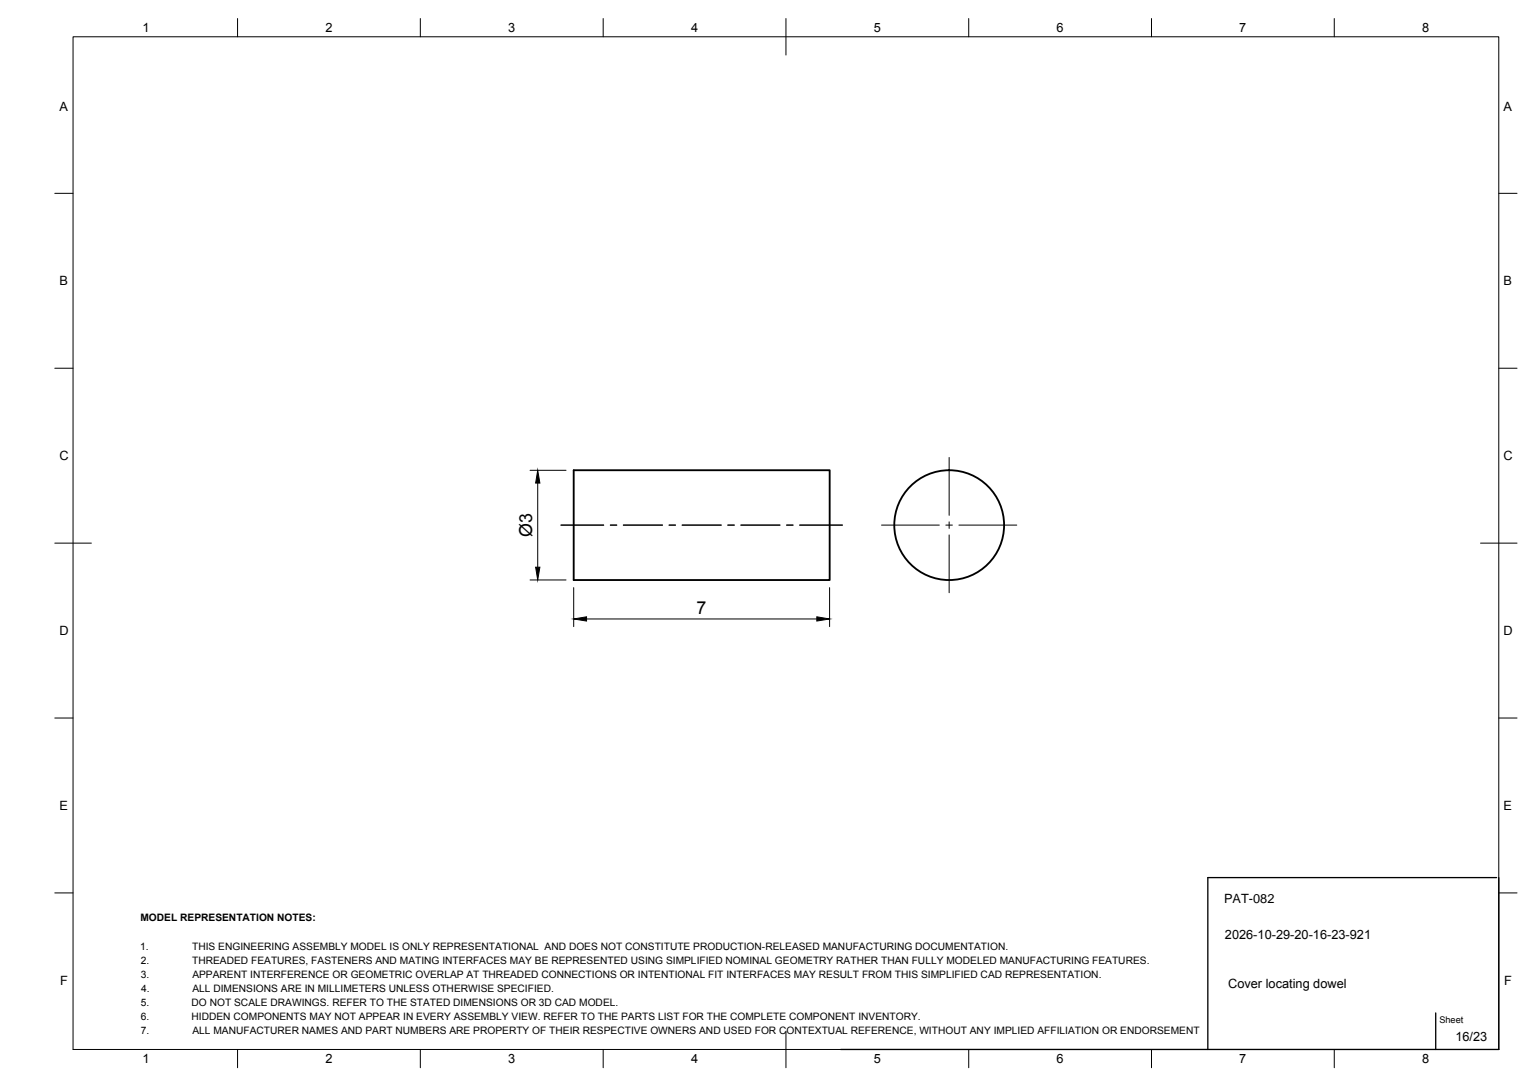
ISO-10303-21;
HEADER;
/* Generated by software containing ST-Developer
 * from STEP Tools, Inc. (www.steptools.com) 
 */

FILE_DESCRIPTION(
/* description */ ('PAT-082'),
/* implementation_level */ '2;1');

FILE_NAME(
/* name */ 'Cover locating dowel.step',
/* time_stamp */ '2026-10-29T20:16:13-07:00',
/* author */ (''),
/* organization */ (''),
/* preprocessor_version */ 'ST-DEVELOPER v20.2',
/* originating_system */ 'Autodesk Translation Framework v15.17.0.0',
/* authorisation */ '');

FILE_SCHEMA (('AUTOMOTIVE_DESIGN { 1 0 10303 214 3 1 1 }'));
ENDSEC;

DATA;
#10=MECHANICAL_DESIGN_GEOMETRIC_PRESENTATION_REPRESENTATION('',(#254),#8266);
#210=SHAPE_REPRESENTATION_RELATIONSHIP('SRR','None',#8372,#232);
#232=ADVANCED_BREP_SHAPE_REPRESENTATION('',(#276),#8256);
#254=STYLED_ITEM('',(#8530),#276);
#276=MANIFOLD_SOLID_BREP('Body1',#4594);
#504=PLANE('',#5182);
#505=PLANE('',#5183);
#741=FACE_OUTER_BOUND('',#1114,.T.);
#742=FACE_OUTER_BOUND('',#1115,.T.);
#743=FACE_OUTER_BOUND('',#1116,.T.);
#1114=EDGE_LOOP('',(#3842,#3843,#3844,#3845));
#1115=EDGE_LOOP('',(#3846));
#1116=EDGE_LOOP('',(#3847));
#1455=LINE('',#7761,#1810);
#1810=VECTOR('',#6266,0.15);
#2091=CIRCLE('',#5180,0.15);
#2092=CIRCLE('',#5181,0.15);
#2397=VERTEX_POINT('',#7758);
#2398=VERTEX_POINT('',#7760);
#2897=EDGE_CURVE('',#2397,#2397,#2091,.T.);
#2898=EDGE_CURVE('',#2397,#2398,#1455,.T.);
#2899=EDGE_CURVE('',#2398,#2398,#2092,.T.);
#3842=ORIENTED_EDGE('',*,*,#2897,.F.);
#3843=ORIENTED_EDGE('',*,*,#2898,.T.);
#3844=ORIENTED_EDGE('',*,*,#2899,.T.);
#3845=ORIENTED_EDGE('',*,*,#2898,.F.);
#3846=ORIENTED_EDGE('',*,*,#2897,.T.);
#3847=ORIENTED_EDGE('',*,*,#2899,.F.);
#4290=CYLINDRICAL_SURFACE('',#5179,0.15);
#4480=ADVANCED_FACE('',(#741),#4290,.T.);
#4481=ADVANCED_FACE('',(#742),#504,.T.);
#4482=ADVANCED_FACE('',(#743),#505,.F.);
#4594=CLOSED_SHELL('',(#4480,#4481,#4482));
#5178=AXIS2_PLACEMENT_3D('',#7756,#6260,#6261);
#5179=AXIS2_PLACEMENT_3D('',#7757,#6262,#6263);
#5180=AXIS2_PLACEMENT_3D('',#7759,#6264,#6265);
#5181=AXIS2_PLACEMENT_3D('',#7762,#6267,#6268);
#5182=AXIS2_PLACEMENT_3D('',#7763,#6269,#6270);
#5183=AXIS2_PLACEMENT_3D('',#7764,#6271,#6272);
#6260=DIRECTION('axis',(0.,0.,1.));
#6261=DIRECTION('refdir',(1.,0.,0.));
#6262=DIRECTION('center_axis',(0.,0.,1.));
#6263=DIRECTION('ref_axis',(1.,0.,0.));
#6264=DIRECTION('center_axis',(0.,0.,1.));
#6265=DIRECTION('ref_axis',(1.,0.,0.));
#6266=DIRECTION('',(0.,0.,-1.));
#6267=DIRECTION('center_axis',(0.,0.,1.));
#6268=DIRECTION('ref_axis',(1.,0.,0.));
#6269=DIRECTION('center_axis',(0.,0.,1.));
#6270=DIRECTION('ref_axis',(1.,0.,0.));
#6271=DIRECTION('center_axis',(0.,0.,1.));
#6272=DIRECTION('ref_axis',(1.,0.,0.));
#7756=CARTESIAN_POINT('',(0.,0.,0.));
#7757=CARTESIAN_POINT('Origin',(-5.,0.,1.6));
#7758=CARTESIAN_POINT('',(-5.15,-1.83697019872103E-17,2.3));
#7759=CARTESIAN_POINT('Origin',(-5.,0.,2.3));
#7760=CARTESIAN_POINT('',(-5.15,-1.83697019872103E-17,1.6));
#7761=CARTESIAN_POINT('',(-5.15,-1.83697019872103E-17,1.6));
#7762=CARTESIAN_POINT('Origin',(-5.,0.,1.6));
#7763=CARTESIAN_POINT('Origin',(-5.,0.,2.3));
#7764=CARTESIAN_POINT('Origin',(-5.,0.,1.6));
#8231=UNCERTAINTY_MEASURE_WITH_UNIT(LENGTH_MEASURE(0.001),#8267,
'DISTANCE_ACCURACY_VALUE',
'Maximum model space distance between geometric entities at asserted c
onnectivities');
#8241=UNCERTAINTY_MEASURE_WITH_UNIT(LENGTH_MEASURE(0.001),#8267,
'DISTANCE_ACCURACY_VALUE',
'Maximum model space distance between geometric entities at asserted c
onnectivities');
#8256=(
GEOMETRIC_REPRESENTATION_CONTEXT(3)
GLOBAL_UNCERTAINTY_ASSIGNED_CONTEXT((#8231))
GLOBAL_UNIT_ASSIGNED_CONTEXT((#8267,#8269,#8270))
REPRESENTATION_CONTEXT('','3D')
);
#8266=(
GEOMETRIC_REPRESENTATION_CONTEXT(3)
GLOBAL_UNCERTAINTY_ASSIGNED_CONTEXT((#8241))
GLOBAL_UNIT_ASSIGNED_CONTEXT((#8267,#8269,#8270))
REPRESENTATION_CONTEXT('','3D')
);
#8267=(
LENGTH_UNIT()
NAMED_UNIT(*)
SI_UNIT(.CENTI.,.METRE.)
);
#8269=(
NAMED_UNIT(*)
PLANE_ANGLE_UNIT()
SI_UNIT($,.RADIAN.)
);
#8270=(
NAMED_UNIT(*)
SI_UNIT($,.STERADIAN.)
SOLID_ANGLE_UNIT()
);
#8285=SHAPE_DEFINITION_REPRESENTATION(#8309,#8372);
#8309=PRODUCT_DEFINITION_SHAPE('',$,#8397);
#8372=SHAPE_REPRESENTATION('',(#5178),#8256);
#8382=PRODUCT_DEFINITION_CONTEXT('part definition',#8456,'design');
#8397=PRODUCT_DEFINITION('Cover locating dowel',
'Cover locating dowel',#8421,#8382);
#8421=PRODUCT_DEFINITION_FORMATION('',$,#8472);
#8456=APPLICATION_CONTEXT(
'Core Data for Automotive Mechanical Design Process');
#8457=PRODUCT_CONTEXT('part definition',#8456,'mechanical');
#8472=PRODUCT('Cover locating dowel','Cover locating dowel',
'Cover locating dowel',(#8457));
#8524=COLOUR_RGB('Sky Blue',0.24,0.69,0.87);
#8525=FILL_AREA_STYLE_COLOUR('',#8524);
#8526=FILL_AREA_STYLE('',(#8525));
#8527=SURFACE_STYLE_FILL_AREA(#8526);
#8528=SURFACE_SIDE_STYLE('',(#8527));
#8529=SURFACE_STYLE_USAGE(.BOTH.,#8528);
#8530=PRESENTATION_STYLE_ASSIGNMENT((#8529));
ENDSEC;
END-ISO-10303-21;
